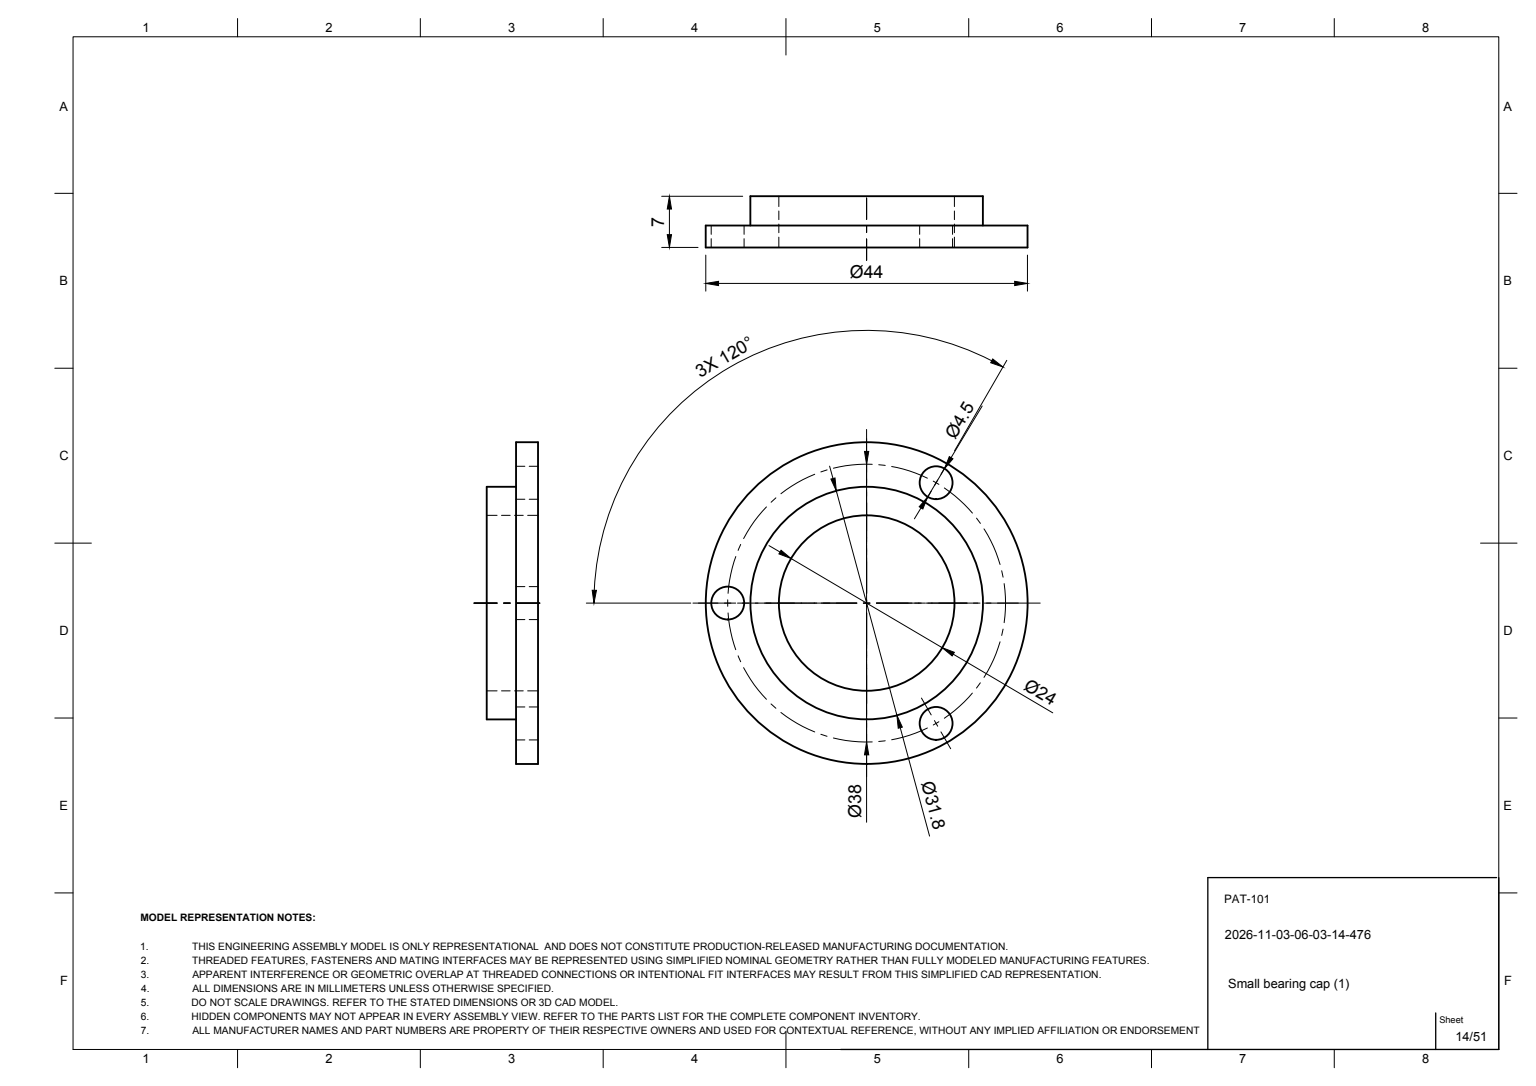
ISO-10303-21;
HEADER;
/* Generated by software containing ST-Developer
 * from STEP Tools, Inc. (www.steptools.com) 
 */

FILE_DESCRIPTION(
/* description */ ('Spur gear reduction stage 2-1 on bearing plates'),
/* implementation_level */ '2;1');

FILE_NAME(
/* name */ 'Small bearing cap (1).step',
/* time_stamp */ '2026-10-28T03:22:07-07:00',
/* author */ (''),
/* organization */ (''),
/* preprocessor_version */ 'ST-DEVELOPER v20.2',
/* originating_system */ 'Autodesk Translation Framework v15.17.0.0',
/* authorisation */ '');

FILE_SCHEMA (('AUTOMOTIVE_DESIGN { 1 0 10303 214 3 1 1 }'));
ENDSEC;

DATA;
#10=MECHANICAL_DESIGN_GEOMETRIC_PRESENTATION_REPRESENTATION('',(#956),#53909);
#870=SHAPE_REPRESENTATION_RELATIONSHIP('SRR','None',#54097,#913);
#913=ADVANCED_BREP_SHAPE_REPRESENTATION('',(#1014),#53871);
#956=STYLED_ITEM('',(#54397),#1014);
#1014=MANIFOLD_SOLID_BREP('Body1',#11280);
#1158=FACE_BOUND('',#2366,.T.);
#1159=FACE_BOUND('',#2370,.T.);
#1160=FACE_BOUND('',#2371,.T.);
#1161=FACE_BOUND('',#2372,.T.);
#1162=FACE_BOUND('',#2373,.T.);
#1163=FACE_BOUND('',#2375,.T.);
#1164=FACE_BOUND('',#2376,.T.);
#1165=FACE_BOUND('',#2377,.T.);
#1166=FACE_BOUND('',#2378,.T.);
#1286=PLANE('',#12070);
#1287=PLANE('',#12077);
#1288=PLANE('',#12078);
#1615=FACE_OUTER_BOUND('',#2361,.T.);
#1616=FACE_OUTER_BOUND('',#2362,.T.);
#1617=FACE_OUTER_BOUND('',#2363,.T.);
#1618=FACE_OUTER_BOUND('',#2364,.T.);
#1619=FACE_OUTER_BOUND('',#2365,.T.);
#1620=FACE_OUTER_BOUND('',#2367,.T.);
#1621=FACE_OUTER_BOUND('',#2368,.T.);
#1622=FACE_OUTER_BOUND('',#2369,.T.);
#1623=FACE_OUTER_BOUND('',#2374,.T.);
#2361=EDGE_LOOP('',(#7808,#7809,#7810,#7811));
#2362=EDGE_LOOP('',(#7812,#7813,#7814,#7815));
#2363=EDGE_LOOP('',(#7816,#7817,#7818,#7819));
#2364=EDGE_LOOP('',(#7820,#7821,#7822,#7823));
#2365=EDGE_LOOP('',(#7824));
#2366=EDGE_LOOP('',(#7825));
#2367=EDGE_LOOP('',(#7826,#7827,#7828,#7829));
#2368=EDGE_LOOP('',(#7830,#7831,#7832,#7833));
#2369=EDGE_LOOP('',(#7834));
#2370=EDGE_LOOP('',(#7835));
#2371=EDGE_LOOP('',(#7836));
#2372=EDGE_LOOP('',(#7837));
#2373=EDGE_LOOP('',(#7838));
#2374=EDGE_LOOP('',(#7839));
#2375=EDGE_LOOP('',(#7840));
#2376=EDGE_LOOP('',(#7841));
#2377=EDGE_LOOP('',(#7842));
#2378=EDGE_LOOP('',(#7843));
#3077=LINE('',#16483,#3718);
#3078=LINE('',#16489,#3719);
#3079=LINE('',#16495,#3720);
#3080=LINE('',#16501,#3721);
#3081=LINE('',#16509,#3722);
#3082=LINE('',#16514,#3723);
#3718=VECTOR('',#13590,0.225);
#3719=VECTOR('',#13597,0.225);
#3720=VECTOR('',#13604,0.225);
#3721=VECTOR('',#13611,1.59);
#3722=VECTOR('',#13622,1.2);
#3723=VECTOR('',#13627,2.2);
#4387=CIRCLE('',#12059,0.225);
#4388=CIRCLE('',#12060,0.225);
#4389=CIRCLE('',#12062,0.225);
#4390=CIRCLE('',#12063,0.225);
#4391=CIRCLE('',#12065,0.225);
#4392=CIRCLE('',#12066,0.225);
#4393=CIRCLE('',#12068,1.59);
#4394=CIRCLE('',#12069,1.59);
#4395=CIRCLE('',#12071,1.2);
#4396=CIRCLE('',#12073,1.2);
#4397=CIRCLE('',#12075,2.2);
#4398=CIRCLE('',#12076,2.2);
#4936=VERTEX_POINT('',#16480);
#4937=VERTEX_POINT('',#16482);
#4938=VERTEX_POINT('',#16486);
#4939=VERTEX_POINT('',#16488);
#4940=VERTEX_POINT('',#16492);
#4941=VERTEX_POINT('',#16494);
#4942=VERTEX_POINT('',#16498);
#4943=VERTEX_POINT('',#16500);
#4944=VERTEX_POINT('',#16504);
#4945=VERTEX_POINT('',#16507);
#4946=VERTEX_POINT('',#16511);
#4947=VERTEX_POINT('',#16513);
#6046=EDGE_CURVE('',#4936,#4936,#4387,.T.);
#6047=EDGE_CURVE('',#4936,#4937,#3077,.T.);
#6048=EDGE_CURVE('',#4937,#4937,#4388,.T.);
#6049=EDGE_CURVE('',#4938,#4938,#4389,.T.);
#6050=EDGE_CURVE('',#4938,#4939,#3078,.T.);
#6051=EDGE_CURVE('',#4939,#4939,#4390,.T.);
#6052=EDGE_CURVE('',#4940,#4940,#4391,.T.);
#6053=EDGE_CURVE('',#4940,#4941,#3079,.T.);
#6054=EDGE_CURVE('',#4941,#4941,#4392,.T.);
#6055=EDGE_CURVE('',#4942,#4942,#4393,.T.);
#6056=EDGE_CURVE('',#4942,#4943,#3080,.T.);
#6057=EDGE_CURVE('',#4943,#4943,#4394,.T.);
#6058=EDGE_CURVE('',#4944,#4944,#4395,.T.);
#6059=EDGE_CURVE('',#4945,#4945,#4396,.T.);
#6060=EDGE_CURVE('',#4945,#4944,#3081,.T.);
#6061=EDGE_CURVE('',#4946,#4946,#4397,.T.);
#6062=EDGE_CURVE('',#4946,#4947,#3082,.T.);
#6063=EDGE_CURVE('',#4947,#4947,#4398,.T.);
#7808=ORIENTED_EDGE('',*,*,#6046,.F.);
#7809=ORIENTED_EDGE('',*,*,#6047,.T.);
#7810=ORIENTED_EDGE('',*,*,#6048,.F.);
#7811=ORIENTED_EDGE('',*,*,#6047,.F.);
#7812=ORIENTED_EDGE('',*,*,#6049,.F.);
#7813=ORIENTED_EDGE('',*,*,#6050,.T.);
#7814=ORIENTED_EDGE('',*,*,#6051,.F.);
#7815=ORIENTED_EDGE('',*,*,#6050,.F.);
#7816=ORIENTED_EDGE('',*,*,#6052,.F.);
#7817=ORIENTED_EDGE('',*,*,#6053,.T.);
#7818=ORIENTED_EDGE('',*,*,#6054,.F.);
#7819=ORIENTED_EDGE('',*,*,#6053,.F.);
#7820=ORIENTED_EDGE('',*,*,#6055,.F.);
#7821=ORIENTED_EDGE('',*,*,#6056,.T.);
#7822=ORIENTED_EDGE('',*,*,#6057,.T.);
#7823=ORIENTED_EDGE('',*,*,#6056,.F.);
#7824=ORIENTED_EDGE('',*,*,#6057,.F.);
#7825=ORIENTED_EDGE('',*,*,#6058,.F.);
#7826=ORIENTED_EDGE('',*,*,#6059,.F.);
#7827=ORIENTED_EDGE('',*,*,#6060,.T.);
#7828=ORIENTED_EDGE('',*,*,#6058,.T.);
#7829=ORIENTED_EDGE('',*,*,#6060,.F.);
#7830=ORIENTED_EDGE('',*,*,#6061,.F.);
#7831=ORIENTED_EDGE('',*,*,#6062,.T.);
#7832=ORIENTED_EDGE('',*,*,#6063,.T.);
#7833=ORIENTED_EDGE('',*,*,#6062,.F.);
#7834=ORIENTED_EDGE('',*,*,#6061,.T.);
#7835=ORIENTED_EDGE('',*,*,#6048,.T.);
#7836=ORIENTED_EDGE('',*,*,#6051,.T.);
#7837=ORIENTED_EDGE('',*,*,#6054,.T.);
#7838=ORIENTED_EDGE('',*,*,#6059,.T.);
#7839=ORIENTED_EDGE('',*,*,#6063,.F.);
#7840=ORIENTED_EDGE('',*,*,#6046,.T.);
#7841=ORIENTED_EDGE('',*,*,#6049,.T.);
#7842=ORIENTED_EDGE('',*,*,#6052,.T.);
#7843=ORIENTED_EDGE('',*,*,#6055,.T.);
#10484=CYLINDRICAL_SURFACE('',#12058,0.225);
#10485=CYLINDRICAL_SURFACE('',#12061,0.225);
#10486=CYLINDRICAL_SURFACE('',#12064,0.225);
#10487=CYLINDRICAL_SURFACE('',#12067,1.59);
#10488=CYLINDRICAL_SURFACE('',#12072,1.2);
#10489=CYLINDRICAL_SURFACE('',#12074,2.2);
#10735=ADVANCED_FACE('',(#1615),#10484,.F.);
#10736=ADVANCED_FACE('',(#1616),#10485,.F.);
#10737=ADVANCED_FACE('',(#1617),#10486,.F.);
#10738=ADVANCED_FACE('',(#1618),#10487,.T.);
#10739=ADVANCED_FACE('',(#1619,#1158),#1286,.F.);
#10740=ADVANCED_FACE('',(#1620),#10488,.F.);
#10741=ADVANCED_FACE('',(#1621),#10489,.T.);
#10742=ADVANCED_FACE('',(#1622,#1159,#1160,#1161,#1162),#1287,.T.);
#10743=ADVANCED_FACE('',(#1623,#1163,#1164,#1165,#1166),#1288,.F.);
#11280=CLOSED_SHELL('',(#10735,#10736,#10737,#10738,#10739,#10740,#10741,
#10742,#10743));
#12057=AXIS2_PLACEMENT_3D('',#16478,#13584,#13585);
#12058=AXIS2_PLACEMENT_3D('',#16479,#13586,#13587);
#12059=AXIS2_PLACEMENT_3D('',#16481,#13588,#13589);
#12060=AXIS2_PLACEMENT_3D('',#16484,#13591,#13592);
#12061=AXIS2_PLACEMENT_3D('',#16485,#13593,#13594);
#12062=AXIS2_PLACEMENT_3D('',#16487,#13595,#13596);
#12063=AXIS2_PLACEMENT_3D('',#16490,#13598,#13599);
#12064=AXIS2_PLACEMENT_3D('',#16491,#13600,#13601);
#12065=AXIS2_PLACEMENT_3D('',#16493,#13602,#13603);
#12066=AXIS2_PLACEMENT_3D('',#16496,#13605,#13606);
#12067=AXIS2_PLACEMENT_3D('',#16497,#13607,#13608);
#12068=AXIS2_PLACEMENT_3D('',#16499,#13609,#13610);
#12069=AXIS2_PLACEMENT_3D('',#16502,#13612,#13613);
#12070=AXIS2_PLACEMENT_3D('',#16503,#13614,#13615);
#12071=AXIS2_PLACEMENT_3D('',#16505,#13616,#13617);
#12072=AXIS2_PLACEMENT_3D('',#16506,#13618,#13619);
#12073=AXIS2_PLACEMENT_3D('',#16508,#13620,#13621);
#12074=AXIS2_PLACEMENT_3D('',#16510,#13623,#13624);
#12075=AXIS2_PLACEMENT_3D('',#16512,#13625,#13626);
#12076=AXIS2_PLACEMENT_3D('',#16515,#13628,#13629);
#12077=AXIS2_PLACEMENT_3D('',#16516,#13630,#13631);
#12078=AXIS2_PLACEMENT_3D('',#16517,#13632,#13633);
#13584=DIRECTION('axis',(0.,0.,1.));
#13585=DIRECTION('refdir',(1.,0.,0.));
#13586=DIRECTION('center_axis',(0.,1.,0.));
#13587=DIRECTION('ref_axis',(1.,0.,0.));
#13588=DIRECTION('center_axis',(0.,1.,0.));
#13589=DIRECTION('ref_axis',(1.,0.,0.));
#13590=DIRECTION('',(0.,1.,0.));
#13591=DIRECTION('center_axis',(0.,-1.,0.));
#13592=DIRECTION('ref_axis',(1.,0.,0.));
#13593=DIRECTION('center_axis',(0.,1.,0.));
#13594=DIRECTION('ref_axis',(1.,0.,0.));
#13595=DIRECTION('center_axis',(0.,1.,0.));
#13596=DIRECTION('ref_axis',(1.,0.,0.));
#13597=DIRECTION('',(0.,1.,0.));
#13598=DIRECTION('center_axis',(0.,-1.,0.));
#13599=DIRECTION('ref_axis',(1.,0.,0.));
#13600=DIRECTION('center_axis',(0.,1.,0.));
#13601=DIRECTION('ref_axis',(1.,0.,0.));
#13602=DIRECTION('center_axis',(0.,1.,0.));
#13603=DIRECTION('ref_axis',(1.,0.,0.));
#13604=DIRECTION('',(0.,1.,0.));
#13605=DIRECTION('center_axis',(0.,-1.,0.));
#13606=DIRECTION('ref_axis',(1.,0.,0.));
#13607=DIRECTION('center_axis',(0.,1.,0.));
#13608=DIRECTION('ref_axis',(1.,0.,0.));
#13609=DIRECTION('center_axis',(0.,1.,0.));
#13610=DIRECTION('ref_axis',(1.,0.,0.));
#13611=DIRECTION('',(0.,-1.,0.));
#13612=DIRECTION('center_axis',(0.,1.,0.));
#13613=DIRECTION('ref_axis',(1.,0.,0.));
#13614=DIRECTION('center_axis',(0.,1.,0.));
#13615=DIRECTION('ref_axis',(1.,0.,0.));
#13616=DIRECTION('center_axis',(0.,-1.,0.));
#13617=DIRECTION('ref_axis',(1.,0.,0.));
#13618=DIRECTION('center_axis',(0.,1.,0.));
#13619=DIRECTION('ref_axis',(1.,0.,0.));
#13620=DIRECTION('center_axis',(0.,-1.,0.));
#13621=DIRECTION('ref_axis',(1.,0.,0.));
#13622=DIRECTION('',(0.,-1.,0.));
#13623=DIRECTION('center_axis',(0.,1.,0.));
#13624=DIRECTION('ref_axis',(1.,0.,0.));
#13625=DIRECTION('center_axis',(0.,1.,0.));
#13626=DIRECTION('ref_axis',(1.,0.,0.));
#13627=DIRECTION('',(0.,-1.,0.));
#13628=DIRECTION('center_axis',(0.,1.,0.));
#13629=DIRECTION('ref_axis',(1.,0.,0.));
#13630=DIRECTION('center_axis',(0.,1.,0.));
#13631=DIRECTION('ref_axis',(1.,0.,0.));
#13632=DIRECTION('center_axis',(0.,1.,0.));
#13633=DIRECTION('ref_axis',(1.,0.,0.));
#16478=CARTESIAN_POINT('',(0.,0.,0.));
#16479=CARTESIAN_POINT('Origin',(1.16341445918999E-16,4.3,6.9));
#16480=CARTESIAN_POINT('',(-0.225,4.4,6.9));
#16481=CARTESIAN_POINT('Origin',(1.16341445918999E-16,4.4,6.9));
#16482=CARTESIAN_POINT('',(-0.225,4.7,6.9));
#16483=CARTESIAN_POINT('',(-0.225,4.3,6.9));
#16484=CARTESIAN_POINT('Origin',(1.16341445918999E-16,4.7,6.9));
#16485=CARTESIAN_POINT('Origin',(-1.64544826719043,4.3,4.05));
#16486=CARTESIAN_POINT('',(-1.87044826719043,4.4,4.05));
#16487=CARTESIAN_POINT('Origin',(-1.64544826719043,4.4,4.05));
#16488=CARTESIAN_POINT('',(-1.87044826719043,4.7,4.05));
#16489=CARTESIAN_POINT('',(-1.87044826719043,4.3,4.05));
#16490=CARTESIAN_POINT('Origin',(-1.64544826719043,4.7,4.05));
#16491=CARTESIAN_POINT('Origin',(1.64544826719043,4.3,4.05));
#16492=CARTESIAN_POINT('',(1.42044826719043,4.4,4.05));
#16493=CARTESIAN_POINT('Origin',(1.64544826719043,4.4,4.05));
#16494=CARTESIAN_POINT('',(1.42044826719043,4.7,4.05));
#16495=CARTESIAN_POINT('',(1.42044826719043,4.3,4.05));
#16496=CARTESIAN_POINT('Origin',(1.64544826719043,4.7,4.05));
#16497=CARTESIAN_POINT('Origin',(0.,4.,5.));
#16498=CARTESIAN_POINT('',(-1.59,4.4,5.));
#16499=CARTESIAN_POINT('Origin',(0.,4.4,5.));
#16500=CARTESIAN_POINT('',(-1.59,4.,5.));
#16501=CARTESIAN_POINT('',(-1.59,4.,5.));
#16502=CARTESIAN_POINT('Origin',(0.,4.,5.));
#16503=CARTESIAN_POINT('Origin',(0.,4.,5.));
#16504=CARTESIAN_POINT('',(-1.2,4.,5.));
#16505=CARTESIAN_POINT('Origin',(0.,4.,5.));
#16506=CARTESIAN_POINT('Origin',(0.,4.4,5.));
#16507=CARTESIAN_POINT('',(-1.2,4.7,5.));
#16508=CARTESIAN_POINT('Origin',(0.,4.7,5.));
#16509=CARTESIAN_POINT('',(-1.2,4.4,5.));
#16510=CARTESIAN_POINT('Origin',(0.,4.4,5.));
#16511=CARTESIAN_POINT('',(-2.2,4.7,5.));
#16512=CARTESIAN_POINT('Origin',(0.,4.7,5.));
#16513=CARTESIAN_POINT('',(-2.2,4.4,5.));
#16514=CARTESIAN_POINT('',(-2.2,4.4,5.));
#16515=CARTESIAN_POINT('Origin',(0.,4.4,5.));
#16516=CARTESIAN_POINT('Origin',(0.,4.7,5.));
#16517=CARTESIAN_POINT('Origin',(0.,4.4,5.));
#53821=UNCERTAINTY_MEASURE_WITH_UNIT(LENGTH_MEASURE(0.001),#53910,
'DISTANCE_ACCURACY_VALUE',
'Maximum model space distance between geometric entities at asserted c
onnectivities');
#53859=UNCERTAINTY_MEASURE_WITH_UNIT(LENGTH_MEASURE(0.001),#53910,
'DISTANCE_ACCURACY_VALUE',
'Maximum model space distance between geometric entities at asserted c
onnectivities');
#53871=(
GEOMETRIC_REPRESENTATION_CONTEXT(3)
GLOBAL_UNCERTAINTY_ASSIGNED_CONTEXT((#53821))
GLOBAL_UNIT_ASSIGNED_CONTEXT((#53910,#53912,#53913))
REPRESENTATION_CONTEXT('','3D')
);
#53909=(
GEOMETRIC_REPRESENTATION_CONTEXT(3)
GLOBAL_UNCERTAINTY_ASSIGNED_CONTEXT((#53859))
GLOBAL_UNIT_ASSIGNED_CONTEXT((#53910,#53912,#53913))
REPRESENTATION_CONTEXT('','3D')
);
#53910=(
LENGTH_UNIT()
NAMED_UNIT(*)
SI_UNIT(.CENTI.,.METRE.)
);
#53912=(
NAMED_UNIT(*)
PLANE_ANGLE_UNIT()
SI_UNIT($,.RADIAN.)
);
#53913=(
NAMED_UNIT(*)
SI_UNIT($,.STERADIAN.)
SOLID_ANGLE_UNIT()
);
#53925=SHAPE_DEFINITION_REPRESENTATION(#53974,#54097);
#53974=PRODUCT_DEFINITION_SHAPE('',$,#54147);
#54097=SHAPE_REPRESENTATION('',(#12057),#53871);
#54135=PRODUCT_DEFINITION_CONTEXT('part definition',#54284,'design');
#54147=PRODUCT_DEFINITION('Small bearing cap (1)','Small bearing cap (1)',
#54196,#54135);
#54196=PRODUCT_DEFINITION_FORMATION('',$,#54297);
#54284=APPLICATION_CONTEXT(
'Core Data for Automotive Mechanical Design Process');
#54285=PRODUCT_CONTEXT('part definition',#54284,'mechanical');
#54297=PRODUCT('Small bearing cap (1)','Small bearing cap (1)',
'Small bearing cap (1)',(#54285));
#54391=COLOUR_RGB('Grey',0.48,0.52,0.57);
#54392=FILL_AREA_STYLE_COLOUR('',#54391);
#54393=FILL_AREA_STYLE('',(#54392));
#54394=SURFACE_STYLE_FILL_AREA(#54393);
#54395=SURFACE_SIDE_STYLE('',(#54394));
#54396=SURFACE_STYLE_USAGE(.BOTH.,#54395);
#54397=PRESENTATION_STYLE_ASSIGNMENT((#54396));
ENDSEC;
END-ISO-10303-21;
